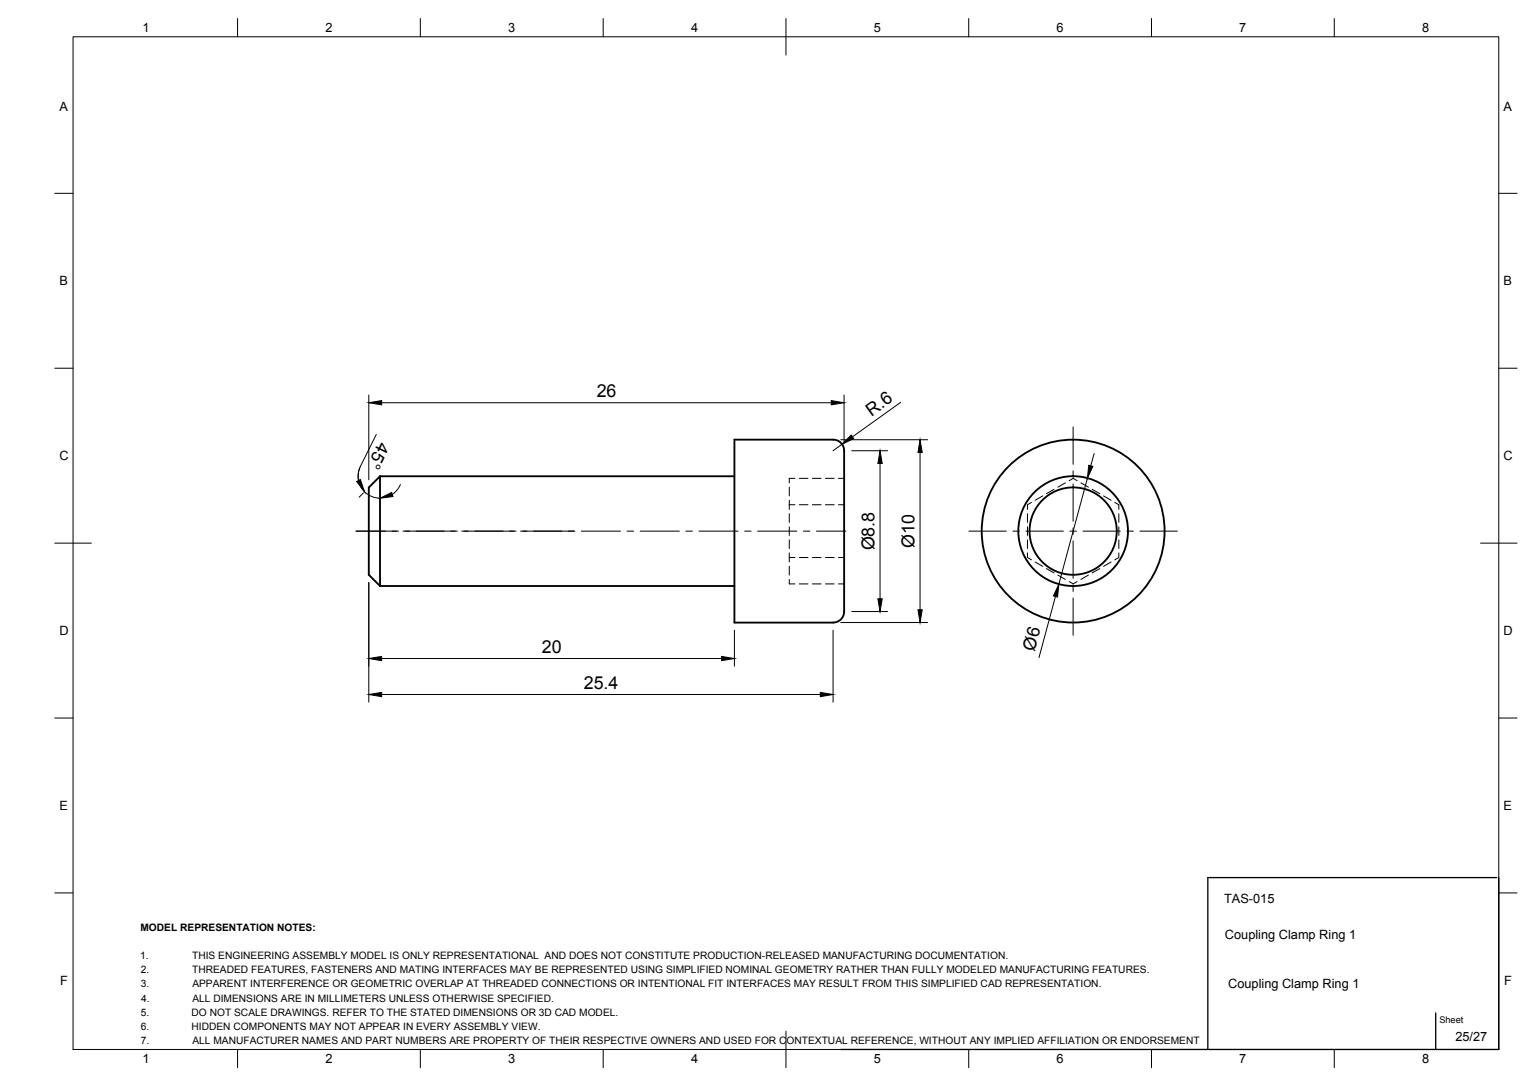
ISO-10303-21;
HEADER;
/* Generated by software containing ST-Developer
 * from STEP Tools, Inc. (www.steptools.com) 
 */

FILE_DESCRIPTION(
/* description */ ('STEP AP214'),
/* implementation_level */ '2;1');

FILE_NAME(
/* name */ 'Coupling Clamp Ring 1.step',
/* time_stamp */ '2026-11-15T14:49:54-08:00',
/* author */ (''),
/* organization */ (''),
/* preprocessor_version */ 'ST-DEVELOPER v20.2',
/* originating_system */ 'Autodesk Translation Framework v15.17.0.0',
/* authorisation */ '');

FILE_SCHEMA (('AUTOMOTIVE_DESIGN { 1 0 10303 214 3 1 1 }'));
ENDSEC;

DATA;
#10=MECHANICAL_DESIGN_GEOMETRIC_PRESENTATION_REPRESENTATION('',(#1122),#66721);
#80=TOROIDAL_SURFACE('',#28228,4.3999999999,0.6);
#555=CONICAL_SURFACE('',#28241,2.693275,0.785398163397448);
#1059=SHAPE_REPRESENTATION_RELATIONSHIP('SRR','None',#66922,#1090);
#1090=ADVANCED_BREP_SHAPE_REPRESENTATION('',(#1157),#66713);
#1122=STYLED_ITEM('',(#67095),#1157);
#1157=MANIFOLD_SOLID_BREP('Body1',#25688);
#1428=FACE_BOUND('',#5166,.T.);
#1429=FACE_BOUND('',#5170,.T.);
#2128=PLANE('',#28223);
#2129=PLANE('',#28231);
#2130=PLANE('',#28232);
#2131=PLANE('',#28233);
#2132=PLANE('',#28234);
#2133=PLANE('',#28235);
#2134=PLANE('',#28236);
#2135=PLANE('',#28237);
#2136=PLANE('',#28238);
#2137=PLANE('',#28239);
#3463=FACE_OUTER_BOUND('',#5165,.T.);
#3464=FACE_OUTER_BOUND('',#5167,.T.);
#3465=FACE_OUTER_BOUND('',#5168,.T.);
#3466=FACE_OUTER_BOUND('',#5169,.T.);
#3467=FACE_OUTER_BOUND('',#5171,.T.);
#3468=FACE_OUTER_BOUND('',#5172,.T.);
#3469=FACE_OUTER_BOUND('',#5173,.T.);
#3470=FACE_OUTER_BOUND('',#5174,.T.);
#3471=FACE_OUTER_BOUND('',#5175,.T.);
#3472=FACE_OUTER_BOUND('',#5176,.T.);
#3473=FACE_OUTER_BOUND('',#5177,.T.);
#3474=FACE_OUTER_BOUND('',#5178,.T.);
#3475=FACE_OUTER_BOUND('',#5179,.T.);
#3476=FACE_OUTER_BOUND('',#5180,.T.);
#5165=EDGE_LOOP('',(#22652));
#5166=EDGE_LOOP('',(#22653));
#5167=EDGE_LOOP('',(#22654,#22655,#22656,#22657));
#5168=EDGE_LOOP('',(#22658,#22659,#22660,#22661));
#5169=EDGE_LOOP('',(#22662));
#5170=EDGE_LOOP('',(#22663,#22664,#22665,#22666,#22667,#22668));
#5171=EDGE_LOOP('',(#22669,#22670,#22671,#22672,#22673,#22674));
#5172=EDGE_LOOP('',(#22675,#22676,#22677,#22678));
#5173=EDGE_LOOP('',(#22679,#22680,#22681,#22682));
#5174=EDGE_LOOP('',(#22683,#22684,#22685,#22686));
#5175=EDGE_LOOP('',(#22687,#22688,#22689,#22690));
#5176=EDGE_LOOP('',(#22691,#22692,#22693,#22694));
#5177=EDGE_LOOP('',(#22695,#22696,#22697,#22698));
#5178=EDGE_LOOP('',(#22699));
#5179=EDGE_LOOP('',(#22700,#22701,#22702,#22703));
#5180=EDGE_LOOP('',(#22704,#22705,#22706,#22707));
#7124=LINE('',#65079,#9113);
#7125=LINE('',#65088,#9114);
#7126=LINE('',#65090,#9115);
#7127=LINE('',#65092,#9116);
#7128=LINE('',#65094,#9117);
#7129=LINE('',#65096,#9118);
#7130=LINE('',#65097,#9119);
#7131=LINE('',#65101,#9120);
#7132=LINE('',#65103,#9121);
#7133=LINE('',#65105,#9122);
#7134=LINE('',#65107,#9123);
#7135=LINE('',#65109,#9124);
#7136=LINE('',#65110,#9125);
#7137=LINE('',#65112,#9126);
#7138=LINE('',#65113,#9127);
#7139=LINE('',#65115,#9128);
#7140=LINE('',#65117,#9129);
#7141=LINE('',#65119,#9130);
#7142=LINE('',#65121,#9131);
#7143=LINE('',#65129,#9132);
#7144=LINE('',#65131,#9133);
#9113=VECTOR('',#34769,5.);
#9114=VECTOR('',#34780,1000.);
#9115=VECTOR('',#34781,1000.);
#9116=VECTOR('',#34782,1000.);
#9117=VECTOR('',#34783,1000.);
#9118=VECTOR('',#34784,1000.);
#9119=VECTOR('',#34785,1000.);
#9120=VECTOR('',#34788,1000.);
#9121=VECTOR('',#34789,1000.);
#9122=VECTOR('',#34790,1000.);
#9123=VECTOR('',#34791,1000.);
#9124=VECTOR('',#34792,1000.);
#9125=VECTOR('',#34793,1000.);
#9126=VECTOR('',#34796,1000.);
#9127=VECTOR('',#34797,1000.);
#9128=VECTOR('',#34800,1000.);
#9129=VECTOR('',#34803,1000.);
#9130=VECTOR('',#34806,1000.);
#9131=VECTOR('',#34809,1000.);
#9132=VECTOR('',#34820,2.693275);
#9133=VECTOR('',#34823,3.);
#10445=CIRCLE('',#28224,5.);
#10446=CIRCLE('',#28225,3.);
#10447=CIRCLE('',#28227,5.);
#10448=CIRCLE('',#28229,0.6);
#10449=CIRCLE('',#28230,4.4);
#10450=CIRCLE('',#28240,2.38655);
#10451=CIRCLE('',#28242,3.);
#12603=VERTEX_POINT('',#65073);
#12604=VERTEX_POINT('',#65075);
#12605=VERTEX_POINT('',#65078);
#12606=VERTEX_POINT('',#65082);
#12607=VERTEX_POINT('',#65086);
#12608=VERTEX_POINT('',#65087);
#12609=VERTEX_POINT('',#65089);
#12610=VERTEX_POINT('',#65091);
#12611=VERTEX_POINT('',#65093);
#12612=VERTEX_POINT('',#65095);
#12613=VERTEX_POINT('',#65099);
#12614=VERTEX_POINT('',#65100);
#12615=VERTEX_POINT('',#65102);
#12616=VERTEX_POINT('',#65104);
#12617=VERTEX_POINT('',#65106);
#12618=VERTEX_POINT('',#65108);
#12619=VERTEX_POINT('',#65124);
#12620=VERTEX_POINT('',#65127);
#16019=EDGE_CURVE('',#12603,#12603,#10445,.T.);
#16020=EDGE_CURVE('',#12604,#12604,#10446,.T.);
#16021=EDGE_CURVE('',#12603,#12605,#7124,.T.);
#16022=EDGE_CURVE('',#12605,#12605,#10447,.T.);
#16023=EDGE_CURVE('',#12605,#12606,#10448,.T.);
#16024=EDGE_CURVE('',#12606,#12606,#10449,.T.);
#16025=EDGE_CURVE('',#12607,#12608,#7125,.T.);
#16026=EDGE_CURVE('',#12608,#12609,#7126,.T.);
#16027=EDGE_CURVE('',#12609,#12610,#7127,.T.);
#16028=EDGE_CURVE('',#12610,#12611,#7128,.T.);
#16029=EDGE_CURVE('',#12611,#12612,#7129,.T.);
#16030=EDGE_CURVE('',#12612,#12607,#7130,.T.);
#16031=EDGE_CURVE('',#12613,#12614,#7131,.T.);
#16032=EDGE_CURVE('',#12614,#12615,#7132,.T.);
#16033=EDGE_CURVE('',#12615,#12616,#7133,.T.);
#16034=EDGE_CURVE('',#12616,#12617,#7134,.T.);
#16035=EDGE_CURVE('',#12617,#12618,#7135,.T.);
#16036=EDGE_CURVE('',#12618,#12613,#7136,.T.);
#16037=EDGE_CURVE('',#12609,#12618,#7137,.T.);
#16038=EDGE_CURVE('',#12608,#12613,#7138,.T.);
#16039=EDGE_CURVE('',#12610,#12617,#7139,.T.);
#16040=EDGE_CURVE('',#12611,#12616,#7140,.T.);
#16041=EDGE_CURVE('',#12612,#12615,#7141,.T.);
#16042=EDGE_CURVE('',#12607,#12614,#7142,.T.);
#16043=EDGE_CURVE('',#12619,#12619,#10450,.T.);
#16044=EDGE_CURVE('',#12620,#12620,#10451,.T.);
#16045=EDGE_CURVE('',#12620,#12619,#7143,.T.);
#16046=EDGE_CURVE('',#12620,#12604,#7144,.T.);
#22652=ORIENTED_EDGE('',*,*,#16019,.T.);
#22653=ORIENTED_EDGE('',*,*,#16020,.T.);
#22654=ORIENTED_EDGE('',*,*,#16019,.F.);
#22655=ORIENTED_EDGE('',*,*,#16021,.T.);
#22656=ORIENTED_EDGE('',*,*,#16022,.T.);
#22657=ORIENTED_EDGE('',*,*,#16021,.F.);
#22658=ORIENTED_EDGE('',*,*,#16022,.F.);
#22659=ORIENTED_EDGE('',*,*,#16023,.T.);
#22660=ORIENTED_EDGE('',*,*,#16024,.T.);
#22661=ORIENTED_EDGE('',*,*,#16023,.F.);
#22662=ORIENTED_EDGE('',*,*,#16024,.F.);
#22663=ORIENTED_EDGE('',*,*,#16025,.T.);
#22664=ORIENTED_EDGE('',*,*,#16026,.T.);
#22665=ORIENTED_EDGE('',*,*,#16027,.T.);
#22666=ORIENTED_EDGE('',*,*,#16028,.T.);
#22667=ORIENTED_EDGE('',*,*,#16029,.T.);
#22668=ORIENTED_EDGE('',*,*,#16030,.T.);
#22669=ORIENTED_EDGE('',*,*,#16031,.T.);
#22670=ORIENTED_EDGE('',*,*,#16032,.T.);
#22671=ORIENTED_EDGE('',*,*,#16033,.T.);
#22672=ORIENTED_EDGE('',*,*,#16034,.T.);
#22673=ORIENTED_EDGE('',*,*,#16035,.T.);
#22674=ORIENTED_EDGE('',*,*,#16036,.T.);
#22675=ORIENTED_EDGE('',*,*,#16036,.F.);
#22676=ORIENTED_EDGE('',*,*,#16037,.F.);
#22677=ORIENTED_EDGE('',*,*,#16026,.F.);
#22678=ORIENTED_EDGE('',*,*,#16038,.T.);
#22679=ORIENTED_EDGE('',*,*,#16035,.F.);
#22680=ORIENTED_EDGE('',*,*,#16039,.F.);
#22681=ORIENTED_EDGE('',*,*,#16027,.F.);
#22682=ORIENTED_EDGE('',*,*,#16037,.T.);
#22683=ORIENTED_EDGE('',*,*,#16034,.F.);
#22684=ORIENTED_EDGE('',*,*,#16040,.F.);
#22685=ORIENTED_EDGE('',*,*,#16028,.F.);
#22686=ORIENTED_EDGE('',*,*,#16039,.T.);
#22687=ORIENTED_EDGE('',*,*,#16033,.F.);
#22688=ORIENTED_EDGE('',*,*,#16041,.F.);
#22689=ORIENTED_EDGE('',*,*,#16029,.F.);
#22690=ORIENTED_EDGE('',*,*,#16040,.T.);
#22691=ORIENTED_EDGE('',*,*,#16032,.F.);
#22692=ORIENTED_EDGE('',*,*,#16042,.F.);
#22693=ORIENTED_EDGE('',*,*,#16030,.F.);
#22694=ORIENTED_EDGE('',*,*,#16041,.T.);
#22695=ORIENTED_EDGE('',*,*,#16031,.F.);
#22696=ORIENTED_EDGE('',*,*,#16038,.F.);
#22697=ORIENTED_EDGE('',*,*,#16025,.F.);
#22698=ORIENTED_EDGE('',*,*,#16042,.T.);
#22699=ORIENTED_EDGE('',*,*,#16043,.T.);
#22700=ORIENTED_EDGE('',*,*,#16044,.T.);
#22701=ORIENTED_EDGE('',*,*,#16045,.T.);
#22702=ORIENTED_EDGE('',*,*,#16043,.F.);
#22703=ORIENTED_EDGE('',*,*,#16045,.F.);
#22704=ORIENTED_EDGE('',*,*,#16044,.F.);
#22705=ORIENTED_EDGE('',*,*,#16046,.T.);
#22706=ORIENTED_EDGE('',*,*,#16020,.F.);
#22707=ORIENTED_EDGE('',*,*,#16046,.F.);
#24144=CYLINDRICAL_SURFACE('',#28226,5.);
#24145=CYLINDRICAL_SURFACE('',#28243,3.);
#25416=ADVANCED_FACE('',(#3463,#1428),#2128,.T.);
#25417=ADVANCED_FACE('',(#3464),#24144,.T.);
#25418=ADVANCED_FACE('',(#3465),#80,.T.);
#25419=ADVANCED_FACE('',(#3466,#1429),#2129,.T.);
#25420=ADVANCED_FACE('',(#3467),#2130,.F.);
#25421=ADVANCED_FACE('',(#3468),#2131,.F.);
#25422=ADVANCED_FACE('',(#3469),#2132,.F.);
#25423=ADVANCED_FACE('',(#3470),#2133,.F.);
#25424=ADVANCED_FACE('',(#3471),#2134,.F.);
#25425=ADVANCED_FACE('',(#3472),#2135,.F.);
#25426=ADVANCED_FACE('',(#3473),#2136,.F.);
#25427=ADVANCED_FACE('',(#3474),#2137,.T.);
#25428=ADVANCED_FACE('',(#3475),#555,.T.);
#25429=ADVANCED_FACE('',(#3476),#24145,.T.);
#25688=CLOSED_SHELL('',(#25416,#25417,#25418,#25419,#25420,#25421,#25422,
#25423,#25424,#25425,#25426,#25427,#25428,#25429));
#28222=AXIS2_PLACEMENT_3D('',#65071,#34759,#34760);
#28223=AXIS2_PLACEMENT_3D('',#65072,#34761,#34762);
#28224=AXIS2_PLACEMENT_3D('',#65074,#34763,#34764);
#28225=AXIS2_PLACEMENT_3D('',#65076,#34765,#34766);
#28226=AXIS2_PLACEMENT_3D('',#65077,#34767,#34768);
#28227=AXIS2_PLACEMENT_3D('',#65080,#34770,#34771);
#28228=AXIS2_PLACEMENT_3D('',#65081,#34772,#34773);
#28229=AXIS2_PLACEMENT_3D('',#65083,#34774,#34775);
#28230=AXIS2_PLACEMENT_3D('',#65084,#34776,#34777);
#28231=AXIS2_PLACEMENT_3D('',#65085,#34778,#34779);
#28232=AXIS2_PLACEMENT_3D('',#65098,#34786,#34787);
#28233=AXIS2_PLACEMENT_3D('',#65111,#34794,#34795);
#28234=AXIS2_PLACEMENT_3D('',#65114,#34798,#34799);
#28235=AXIS2_PLACEMENT_3D('',#65116,#34801,#34802);
#28236=AXIS2_PLACEMENT_3D('',#65118,#34804,#34805);
#28237=AXIS2_PLACEMENT_3D('',#65120,#34807,#34808);
#28238=AXIS2_PLACEMENT_3D('',#65122,#34810,#34811);
#28239=AXIS2_PLACEMENT_3D('',#65123,#34812,#34813);
#28240=AXIS2_PLACEMENT_3D('',#65125,#34814,#34815);
#28241=AXIS2_PLACEMENT_3D('',#65126,#34816,#34817);
#28242=AXIS2_PLACEMENT_3D('',#65128,#34818,#34819);
#28243=AXIS2_PLACEMENT_3D('',#65130,#34821,#34822);
#34759=DIRECTION('axis',(0.,0.,1.));
#34760=DIRECTION('refdir',(1.,0.,0.));
#34761=DIRECTION('center_axis',(0.,0.707106781186548,0.707106781186548));
#34762=DIRECTION('ref_axis',(1.,0.,0.));
#34763=DIRECTION('center_axis',(0.,0.707106781186548,0.707106781186548));
#34764=DIRECTION('ref_axis',(-1.,0.,0.));
#34765=DIRECTION('center_axis',(0.,-0.707106781186548,-0.707106781186548));
#34766=DIRECTION('ref_axis',(-1.,0.,0.));
#34767=DIRECTION('center_axis',(0.,0.707106781186548,0.707106781186548));
#34768=DIRECTION('ref_axis',(-1.,0.,0.));
#34769=DIRECTION('',(0.,-0.707106781186547,-0.707106781186547));
#34770=DIRECTION('center_axis',(0.,0.707106781186548,0.707106781186548));
#34771=DIRECTION('ref_axis',(-1.,0.,0.));
#34772=DIRECTION('center_axis',(0.,0.707106781186548,0.707106781186548));
#34773=DIRECTION('ref_axis',(-1.,0.,0.));
#34774=DIRECTION('center_axis',(-7.85046229357589E-17,0.707106781186548,
-0.707106781186548));
#34775=DIRECTION('ref_axis',(1.,0.,-1.11022302464736E-16));
#34776=DIRECTION('center_axis',(0.,0.707106781186548,0.707106781186548));
#34777=DIRECTION('ref_axis',(-1.,0.,0.));
#34778=DIRECTION('center_axis',(-2.27272746077357E-11,-0.707106781186548,
-0.707106781186548));
#34779=DIRECTION('ref_axis',(-4.86851002232982E-28,-0.707106781186548,0.707106781186548));
#34780=DIRECTION('',(0.,0.707106781186547,-0.707106781186547));
#34781=DIRECTION('',(-0.866025403795548,0.353553390593585,-0.35355339056575));
#34782=DIRECTION('',(-0.866025403795548,-0.35355339056575,0.353553390593585));
#34783=DIRECTION('',(0.,-0.707106781186547,0.707106781186547));
#34784=DIRECTION('',(0.866025403795548,-0.353553390593585,0.35355339056575));
#34785=DIRECTION('',(0.866025403795548,0.35355339056575,-0.353553390593585));
#34786=DIRECTION('center_axis',(0.,0.707106781186547,0.707106781186548));
#34787=DIRECTION('ref_axis',(1.,0.,0.));
#34788=DIRECTION('',(0.,-0.707106781186548,0.707106781186547));
#34789=DIRECTION('',(-0.866025403795548,-0.353553390579667,0.353553390579667));
#34790=DIRECTION('',(-0.866025403795548,0.353553390579667,-0.353553390579667));
#34791=DIRECTION('',(0.,0.707106781186548,-0.707106781186547));
#34792=DIRECTION('',(0.866025403795548,0.353553390579667,-0.353553390579667));
#34793=DIRECTION('',(0.866025403795548,-0.353553390579667,0.353553390579667));
#34794=DIRECTION('center_axis',(0.499999999980758,0.61237243570365,-0.61237243570365));
#34795=DIRECTION('ref_axis',(-0.774596669257382,1.17004406563443E-17,-0.632455532014204));
#34796=DIRECTION('',(0.,0.707106781186547,0.707106781186548));
#34797=DIRECTION('',(0.,0.707106781186547,0.707106781186548));
#34798=DIRECTION('center_axis',(-0.499999999980758,0.61237243570365,-0.61237243570365));
#34799=DIRECTION('ref_axis',(-0.774596669257382,-1.17004406563443E-17,0.632455532014204));
#34800=DIRECTION('',(0.,0.707106781186547,0.707106781186548));
#34801=DIRECTION('center_axis',(-1.,0.,0.));
#34802=DIRECTION('ref_axis',(0.,0.,1.));
#34803=DIRECTION('',(0.,0.707106781186547,0.707106781186548));
#34804=DIRECTION('center_axis',(-0.499999999980758,-0.61237243570365,0.61237243570365));
#34805=DIRECTION('ref_axis',(-0.774596669257382,0.632455532014204,-1.19590756914335E-17));
#34806=DIRECTION('',(0.,0.707106781186547,0.707106781186548));
#34807=DIRECTION('center_axis',(0.499999999980758,-0.61237243570365,0.61237243570365));
#34808=DIRECTION('ref_axis',(-0.774596669257382,-0.632455532014204,1.19590756914335E-17));
#34809=DIRECTION('',(0.,0.707106781186547,0.707106781186548));
#34810=DIRECTION('center_axis',(1.,0.,0.));
#34811=DIRECTION('ref_axis',(0.,1.,0.));
#34812=DIRECTION('center_axis',(0.,0.707106781186548,0.707106781186548));
#34813=DIRECTION('ref_axis',(1.,0.,0.));
#34814=DIRECTION('center_axis',(0.,0.707106781186548,0.707106781186548));
#34815=DIRECTION('ref_axis',(-1.,0.,0.));
#34816=DIRECTION('center_axis',(0.,-0.707106781186548,-0.707106781186548));
#34817=DIRECTION('ref_axis',(-1.,0.,0.));
#34818=DIRECTION('center_axis',(0.,0.707106781186548,0.707106781186548));
#34819=DIRECTION('ref_axis',(-1.,0.,0.));
#34820=DIRECTION('',(-0.707106781186547,0.5,0.5));
#34821=DIRECTION('center_axis',(0.,0.707106781186548,0.707106781186548));
#34822=DIRECTION('ref_axis',(-1.,0.,0.));
#34823=DIRECTION('',(0.,-0.707106781186548,-0.707106781186548));
#65071=CARTESIAN_POINT('',(0.,0.,0.));
#65072=CARTESIAN_POINT('Origin',(-26.5,-22.6274169980807,5.65685424941929));
#65073=CARTESIAN_POINT('',(-19.,-22.6274169980807,5.65685424941929));
#65074=CARTESIAN_POINT('Origin',(-24.,-22.6274169980807,5.65685424941929));
#65075=CARTESIAN_POINT('',(-21.,-22.6274169980807,5.65685424941928));
#65076=CARTESIAN_POINT('Origin',(-24.,-22.6274169980807,5.65685424941928));
#65077=CARTESIAN_POINT('Origin',(-24.,-24.5366053072844,3.74766594021561));
#65078=CARTESIAN_POINT('',(-19.,-26.4457936164881,1.83847763101193));
#65079=CARTESIAN_POINT('',(-19.,-24.5366053072844,3.74766594021561));
#65080=CARTESIAN_POINT('Origin',(-24.,-26.4457936164881,1.83847763101193));
#65081=CARTESIAN_POINT('Origin',(-24.,-26.4457936164174,1.83847763108264));
#65082=CARTESIAN_POINT('',(-19.6,-26.8700576851293,1.41421356237071));
#65083=CARTESIAN_POINT('Origin',(-19.6000000001,-26.4457936164174,1.83847763108264));
#65084=CARTESIAN_POINT('Origin',(-24.,-26.8700576851293,1.41421356237071));
#65085=CARTESIAN_POINT('Origin',(-26.2,-26.8700576851646,1.41421356233536));
#65086=CARTESIAN_POINT('',(-21.5,-27.890678411278,2.434834288578));
#65087=CARTESIAN_POINT('',(-21.5,-25.849436958922,0.393592836222004));
#65088=CARTESIAN_POINT('',(-21.5,-26.8700576852402,1.41421356225982));
#65089=CARTESIAN_POINT('',(-24.,-24.8288162328147,-0.627027889885282));
#65090=CARTESIAN_POINT('',(-23.5750000000476,-25.0023217562335,-0.453522366466486));
#65091=CARTESIAN_POINT('',(-26.5,-25.849436958922,0.393592836222004));
#65092=CARTESIAN_POINT('',(-26.0749999999947,-25.6759314354816,0.220087312781607));
#65093=CARTESIAN_POINT('',(-26.5,-27.890678411278,2.434834288578));
#65094=CARTESIAN_POINT('',(-26.5,-26.6149025036153,1.15905838079568));
#65095=CARTESIAN_POINT('',(-24.,-28.9112991373853,3.45545501468528));
#65096=CARTESIAN_POINT('',(-26.0749999999947,-28.0641839347184,2.60833981201839));
#65097=CARTESIAN_POINT('',(-23.5750000000476,-28.7377936139665,3.28194949126649));
#65098=CARTESIAN_POINT('Origin',(-24.,-24.7487373415404,3.53553390595964));
#65099=CARTESIAN_POINT('',(-21.5,-23.7281166153624,2.51491317978165));
#65100=CARTESIAN_POINT('',(-21.5,-25.7693580677184,4.55615463213764));
#65101=CARTESIAN_POINT('',(-21.5,-25.7693580677184,4.55615463213764));
#65102=CARTESIAN_POINT('',(-24.,-26.7899787938256,5.57677535824492));
#65103=CARTESIAN_POINT('',(-24.,-26.7899787938256,5.57677535824492));
#65104=CARTESIAN_POINT('',(-26.5,-25.7693580677184,4.55615463213764));
#65105=CARTESIAN_POINT('',(-26.5,-25.7693580677184,4.55615463213764));
#65106=CARTESIAN_POINT('',(-26.5,-23.7281166153624,2.51491317978165));
#65107=CARTESIAN_POINT('',(-26.5,-24.7487373415404,3.53553390595964));
#65108=CARTESIAN_POINT('',(-24.,-22.7074958892551,1.49429245367436));
#65109=CARTESIAN_POINT('',(-24.,-22.7074958892551,1.49429245367436));
#65110=CARTESIAN_POINT('',(-21.5,-23.7281166153624,2.51491317978165));
#65111=CARTESIAN_POINT('Origin',(-22.75,-25.3391265958684,-0.116717526831639));
#65112=CARTESIAN_POINT('',(-24.,-24.8288162328147,-0.627027889885282));
#65113=CARTESIAN_POINT('',(-21.5,-25.849436958922,0.393592836222004));
#65114=CARTESIAN_POINT('Origin',(-25.25,-25.3391265958684,-0.116717526831639));
#65115=CARTESIAN_POINT('',(-26.5,-25.849436958922,0.393592836222004));
#65116=CARTESIAN_POINT('Origin',(-26.5,-26.359747322011,0.903903199311002));
#65117=CARTESIAN_POINT('',(-26.5,-27.890678411278,2.434834288578));
#65118=CARTESIAN_POINT('Origin',(-25.25,-28.4009887743316,2.94514465163164));
#65119=CARTESIAN_POINT('',(-24.,-28.9112991373853,3.45545501468528));
#65120=CARTESIAN_POINT('Origin',(-22.75,-28.4009887743316,2.94514465163164));
#65121=CARTESIAN_POINT('',(-21.5,-27.890678411278,2.434834288578));
#65122=CARTESIAN_POINT('Origin',(-21.5,-26.8700576851,1.4142135624));
#65123=CARTESIAN_POINT('Origin',(-25.193275,-8.48528137426905,19.798989873231));
#65124=CARTESIAN_POINT('',(-21.61345,-8.48528137426905,19.7989898732309));
#65125=CARTESIAN_POINT('Origin',(-24.,-8.48528137426905,19.798989873231));
#65126=CARTESIAN_POINT('Origin',(-24.,-8.70216870172849,19.5821025457715));
#65127=CARTESIAN_POINT('',(-21.,-8.91905602918794,19.3652152183121));
#65128=CARTESIAN_POINT('Origin',(-24.,-8.91905602918794,19.3652152183121));
#65129=CARTESIAN_POINT('',(-21.306725,-8.70216870172849,19.5821025457715));
#65130=CARTESIAN_POINT('Origin',(-24.,-15.773236513594,12.511034733906));
#65131=CARTESIAN_POINT('',(-21.,-15.773236513594,12.511034733906));
#66672=UNCERTAINTY_MEASURE_WITH_UNIT(LENGTH_MEASURE(0.01),#66722,
'DISTANCE_ACCURACY_VALUE',
'Maximum model space distance between geometric entities at asserted c
onnectivities');
#66680=UNCERTAINTY_MEASURE_WITH_UNIT(LENGTH_MEASURE(0.01),#66722,
'DISTANCE_ACCURACY_VALUE',
'Maximum model space distance between geometric entities at asserted c
onnectivities');
#66713=(
GEOMETRIC_REPRESENTATION_CONTEXT(3)
GLOBAL_UNCERTAINTY_ASSIGNED_CONTEXT((#66672))
GLOBAL_UNIT_ASSIGNED_CONTEXT((#66722,#66724,#66725))
REPRESENTATION_CONTEXT('','3D')
);
#66721=(
GEOMETRIC_REPRESENTATION_CONTEXT(3)
GLOBAL_UNCERTAINTY_ASSIGNED_CONTEXT((#66680))
GLOBAL_UNIT_ASSIGNED_CONTEXT((#66722,#66724,#66725))
REPRESENTATION_CONTEXT('','3D')
);
#66722=(
LENGTH_UNIT()
NAMED_UNIT(*)
SI_UNIT(.MILLI.,.METRE.)
);
#66724=(
NAMED_UNIT(*)
PLANE_ANGLE_UNIT()
SI_UNIT($,.RADIAN.)
);
#66725=(
NAMED_UNIT(*)
SI_UNIT($,.STERADIAN.)
SOLID_ANGLE_UNIT()
);
#66758=SHAPE_DEFINITION_REPRESENTATION(#66818,#66922);
#66818=PRODUCT_DEFINITION_SHAPE('',$,#66963);
#66922=SHAPE_REPRESENTATION('',(#28222),#66713);
#66930=PRODUCT_DEFINITION_CONTEXT('part definition',#67052,'design');
#66963=PRODUCT_DEFINITION('Coupling Clamp Ring 1',
'Coupling Clamp Ring 1',#67003,#66930);
#67003=PRODUCT_DEFINITION_FORMATION('',$,#67086);
#67052=APPLICATION_CONTEXT(
'Core Data for Automotive Mechanical Design Process');
#67053=PRODUCT_CONTEXT('part definition',#67052,'mechanical');
#67086=PRODUCT('Coupling Clamp Ring 1','Coupling Clamp Ring 1',$,(#67053));
#67095=PRESENTATION_STYLE_ASSIGNMENT((#67097));
#67097=SURFACE_STYLE_USAGE(.BOTH.,#67099);
#67099=SURFACE_SIDE_STYLE('',(#67101));
#67101=SURFACE_STYLE_FILL_AREA(#67103);
#67103=FILL_AREA_STYLE('Opaque(202,209,238)',(#67105));
#67105=FILL_AREA_STYLE_COLOUR('Opaque(202,209,238)',#67107);
#67107=COLOUR_RGB('Opaque(202,209,238)',0.792156862745098,0.819607843137255,
0.933333333333333);
ENDSEC;
END-ISO-10303-21;
